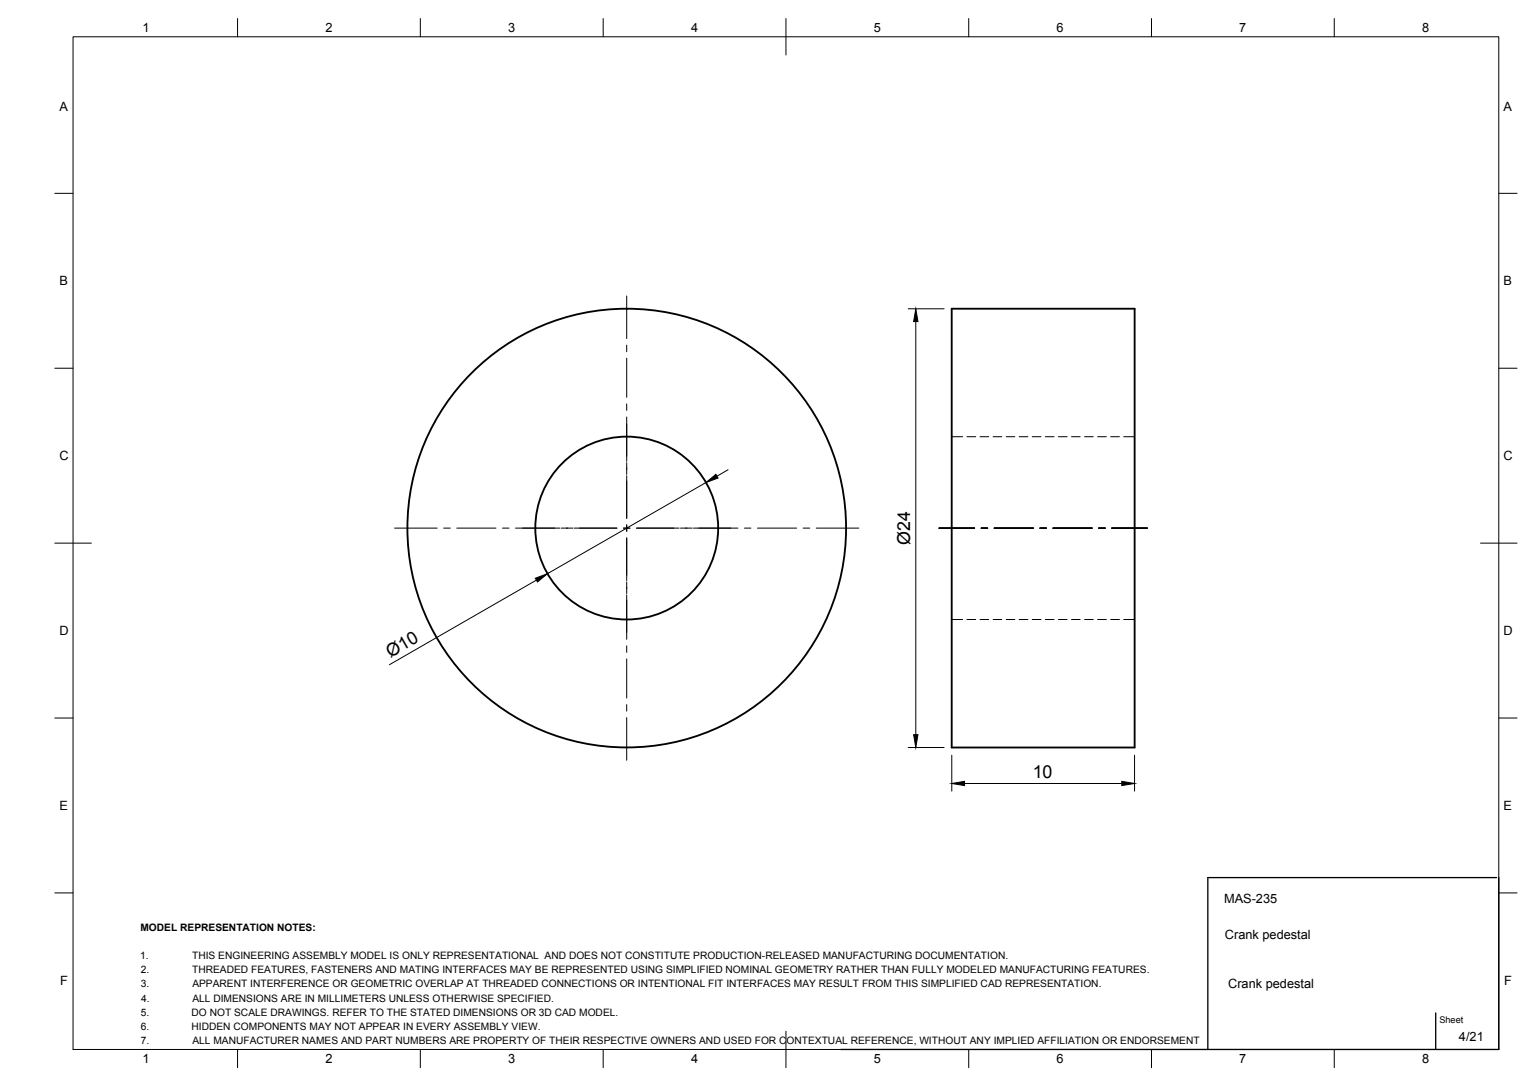
ISO-10303-21;
HEADER;
/* Generated by software containing ST-Developer
 * from STEP Tools, Inc. (www.steptools.com) 
 */

FILE_DESCRIPTION(
/* description */ ('Independent Whitworth quick-return mechanism. Crank radius40, ground-
center spacing80, lever180, connecting rod160, output guide X200. Nomi
nal stroke180 and long/short phase ratio2. Retained guide rods, replac
eable bearing sleeves and captured sliding shoe. No load or production
 rating assigned.'),
/* implementation_level */ '2;1');

FILE_NAME(
/* name */ 'Crank pedestal.step',
/* time_stamp */ '2026-11-09T18:22:56-08:00',
/* author */ (''),
/* organization */ (''),
/* preprocessor_version */ 'ST-DEVELOPER v20.2',
/* originating_system */ 'Autodesk Translation Framework v15.17.0.0',
/* authorisation */ '');

FILE_SCHEMA (('AUTOMOTIVE_DESIGN { 1 0 10303 214 3 1 1 }'));
ENDSEC;

DATA;
#10=MECHANICAL_DESIGN_GEOMETRIC_PRESENTATION_REPRESENTATION('',(#220),#4388);
#180=SHAPE_REPRESENTATION_RELATIONSHIP('SRR','None',#4479,#200);
#200=ADVANCED_BREP_SHAPE_REPRESENTATION('',(#240),#4369);
#220=STYLED_ITEM('',(#4588),#240);
#240=MANIFOLD_SOLID_BREP('Body1',#2325);
#263=FACE_BOUND('',#567,.T.);
#264=FACE_BOUND('',#569,.T.);
#325=PLANE('',#2586);
#326=PLANE('',#2587);
#413=FACE_OUTER_BOUND('',#564,.T.);
#414=FACE_OUTER_BOUND('',#565,.T.);
#415=FACE_OUTER_BOUND('',#566,.T.);
#416=FACE_OUTER_BOUND('',#568,.T.);
#564=EDGE_LOOP('',(#1630,#1631,#1632,#1633));
#565=EDGE_LOOP('',(#1634,#1635,#1636,#1637));
#566=EDGE_LOOP('',(#1638));
#567=EDGE_LOOP('',(#1639));
#568=EDGE_LOOP('',(#1640));
#569=EDGE_LOOP('',(#1641));
#773=LINE('',#3745,#912);
#774=LINE('',#3751,#913);
#912=VECTOR('',#2945,5.);
#913=VECTOR('',#2952,12.);
#1041=CIRCLE('',#2581,5.);
#1042=CIRCLE('',#2582,5.);
#1043=CIRCLE('',#2584,12.);
#1044=CIRCLE('',#2585,12.);
#1171=VERTEX_POINT('',#3742);
#1172=VERTEX_POINT('',#3744);
#1173=VERTEX_POINT('',#3748);
#1174=VERTEX_POINT('',#3750);
#1351=EDGE_CURVE('',#1171,#1171,#1041,.T.);
#1352=EDGE_CURVE('',#1171,#1172,#773,.T.);
#1353=EDGE_CURVE('',#1172,#1172,#1042,.T.);
#1354=EDGE_CURVE('',#1173,#1173,#1043,.T.);
#1355=EDGE_CURVE('',#1173,#1174,#774,.T.);
#1356=EDGE_CURVE('',#1174,#1174,#1044,.T.);
#1630=ORIENTED_EDGE('',*,*,#1351,.F.);
#1631=ORIENTED_EDGE('',*,*,#1352,.T.);
#1632=ORIENTED_EDGE('',*,*,#1353,.T.);
#1633=ORIENTED_EDGE('',*,*,#1352,.F.);
#1634=ORIENTED_EDGE('',*,*,#1354,.F.);
#1635=ORIENTED_EDGE('',*,*,#1355,.T.);
#1636=ORIENTED_EDGE('',*,*,#1356,.T.);
#1637=ORIENTED_EDGE('',*,*,#1355,.F.);
#1638=ORIENTED_EDGE('',*,*,#1354,.T.);
#1639=ORIENTED_EDGE('',*,*,#1351,.T.);
#1640=ORIENTED_EDGE('',*,*,#1356,.F.);
#1641=ORIENTED_EDGE('',*,*,#1353,.F.);
#2118=CYLINDRICAL_SURFACE('',#2580,5.);
#2119=CYLINDRICAL_SURFACE('',#2583,12.);
#2185=ADVANCED_FACE('',(#413),#2118,.F.);
#2186=ADVANCED_FACE('',(#414),#2119,.T.);
#2187=ADVANCED_FACE('',(#415,#263),#325,.T.);
#2188=ADVANCED_FACE('',(#416,#264),#326,.F.);
#2325=CLOSED_SHELL('',(#2185,#2186,#2187,#2188));
#2579=AXIS2_PLACEMENT_3D('',#3740,#2939,#2940);
#2580=AXIS2_PLACEMENT_3D('',#3741,#2941,#2942);
#2581=AXIS2_PLACEMENT_3D('',#3743,#2943,#2944);
#2582=AXIS2_PLACEMENT_3D('',#3746,#2946,#2947);
#2583=AXIS2_PLACEMENT_3D('',#3747,#2948,#2949);
#2584=AXIS2_PLACEMENT_3D('',#3749,#2950,#2951);
#2585=AXIS2_PLACEMENT_3D('',#3752,#2953,#2954);
#2586=AXIS2_PLACEMENT_3D('',#3753,#2955,#2956);
#2587=AXIS2_PLACEMENT_3D('',#3754,#2957,#2958);
#2939=DIRECTION('axis',(0.,0.,1.));
#2940=DIRECTION('refdir',(1.,0.,0.));
#2941=DIRECTION('center_axis',(0.,0.,1.));
#2942=DIRECTION('ref_axis',(1.,0.,0.));
#2943=DIRECTION('center_axis',(0.,0.,-1.));
#2944=DIRECTION('ref_axis',(1.,0.,0.));
#2945=DIRECTION('',(0.,0.,-1.));
#2946=DIRECTION('center_axis',(0.,0.,-1.));
#2947=DIRECTION('ref_axis',(1.,0.,0.));
#2948=DIRECTION('center_axis',(0.,0.,1.));
#2949=DIRECTION('ref_axis',(1.,0.,0.));
#2950=DIRECTION('center_axis',(0.,0.,1.));
#2951=DIRECTION('ref_axis',(1.,0.,0.));
#2952=DIRECTION('',(0.,0.,-1.));
#2953=DIRECTION('center_axis',(0.,0.,1.));
#2954=DIRECTION('ref_axis',(1.,0.,0.));
#2955=DIRECTION('center_axis',(0.,0.,1.));
#2956=DIRECTION('ref_axis',(1.,0.,0.));
#2957=DIRECTION('center_axis',(0.,0.,1.));
#2958=DIRECTION('ref_axis',(1.,0.,0.));
#3740=CARTESIAN_POINT('',(0.,0.,0.));
#3741=CARTESIAN_POINT('Origin',(0.,0.,0.));
#3742=CARTESIAN_POINT('',(-5.,-6.12323399573677E-16,10.));
#3743=CARTESIAN_POINT('Origin',(0.,0.,10.));
#3744=CARTESIAN_POINT('',(-5.,-6.12323399573677E-16,0.));
#3745=CARTESIAN_POINT('',(-5.,-6.12323399573677E-16,0.));
#3746=CARTESIAN_POINT('Origin',(0.,0.,0.));
#3747=CARTESIAN_POINT('Origin',(0.,0.,0.));
#3748=CARTESIAN_POINT('',(-12.,-1.46957615897682E-15,10.));
#3749=CARTESIAN_POINT('Origin',(0.,0.,10.));
#3750=CARTESIAN_POINT('',(-12.,-1.46957615897682E-15,0.));
#3751=CARTESIAN_POINT('',(-12.,-1.46957615897682E-15,0.));
#3752=CARTESIAN_POINT('Origin',(0.,0.,0.));
#3753=CARTESIAN_POINT('Origin',(0.,0.,10.));
#3754=CARTESIAN_POINT('Origin',(0.,0.,0.));
#4347=UNCERTAINTY_MEASURE_WITH_UNIT(LENGTH_MEASURE(0.01),#4389,
'DISTANCE_ACCURACY_VALUE',
'Maximum model space distance between geometric entities at asserted c
onnectivities');
#4366=UNCERTAINTY_MEASURE_WITH_UNIT(LENGTH_MEASURE(0.01),#4389,
'DISTANCE_ACCURACY_VALUE',
'Maximum model space distance between geometric entities at asserted c
onnectivities');
#4369=(
GEOMETRIC_REPRESENTATION_CONTEXT(3)
GLOBAL_UNCERTAINTY_ASSIGNED_CONTEXT((#4347))
GLOBAL_UNIT_ASSIGNED_CONTEXT((#4389,#4391,#4392))
REPRESENTATION_CONTEXT('','3D')
);
#4388=(
GEOMETRIC_REPRESENTATION_CONTEXT(3)
GLOBAL_UNCERTAINTY_ASSIGNED_CONTEXT((#4366))
GLOBAL_UNIT_ASSIGNED_CONTEXT((#4389,#4391,#4392))
REPRESENTATION_CONTEXT('','3D')
);
#4389=(
LENGTH_UNIT()
NAMED_UNIT(*)
SI_UNIT(.MILLI.,.METRE.)
);
#4391=(
NAMED_UNIT(*)
PLANE_ANGLE_UNIT()
SI_UNIT($,.RADIAN.)
);
#4392=(
NAMED_UNIT(*)
SI_UNIT($,.STERADIAN.)
SOLID_ANGLE_UNIT()
);
#4395=SHAPE_DEFINITION_REPRESENTATION(#4416,#4479);
#4416=PRODUCT_DEFINITION_SHAPE('',$,#4501);
#4479=SHAPE_REPRESENTATION('',(#2579),#4369);
#4498=PRODUCT_DEFINITION_CONTEXT('part definition',#4563,'design');
#4501=PRODUCT_DEFINITION('Crank pedestal','Crank pedestal',#4522,#4498);
#4522=PRODUCT_DEFINITION_FORMATION('',$,#4567);
#4563=APPLICATION_CONTEXT(
'Core Data for Automotive Mechanical Design Process');
#4564=PRODUCT_CONTEXT('part definition',#4563,'mechanical');
#4567=PRODUCT('Crank pedestal','Crank pedestal',$,(#4564));
#4588=PRESENTATION_STYLE_ASSIGNMENT((#4602));
#4602=SURFACE_STYLE_USAGE(.BOTH.,#4616);
#4616=SURFACE_SIDE_STYLE('',(#4630));
#4630=SURFACE_STYLE_FILL_AREA(#4644);
#4644=FILL_AREA_STYLE('Support gray',(#4658));
#4658=FILL_AREA_STYLE_COLOUR('Support gray',#4672);
#4672=COLOUR_RGB('Support gray',0.407843137254902,0.447058823529412,0.498039215686275);
ENDSEC;
END-ISO-10303-21;
